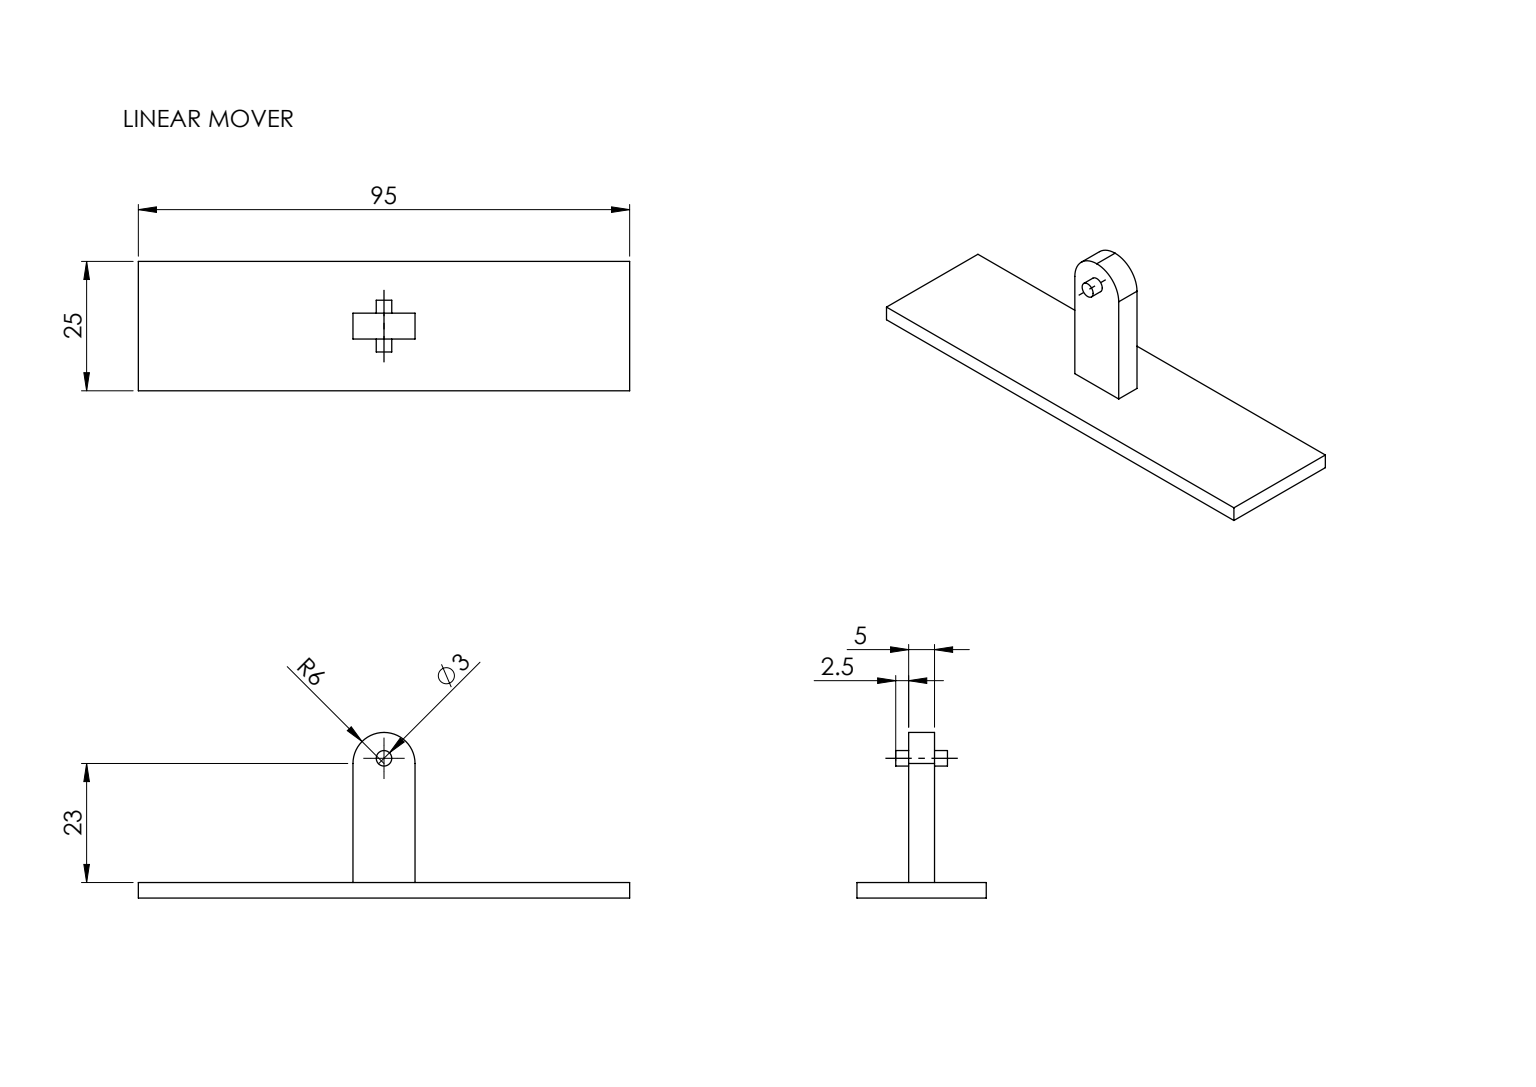
ISO-10303-21;
HEADER;
FILE_DESCRIPTION (('STEP AP214'),
    '1' );
FILE_NAME ('linear mover.step',
    '2026-10-04T07:56:41',
    ( '' ),
    ( '' ),
    'SwSTEP 2.0',
    'SolidWorks 2026',
    '' );
FILE_SCHEMA (( 'AUTOMOTIVE_DESIGN' ));
ENDSEC;

DATA;
#6=DIRECTION ( 'NONE',  ( -1.000000000000000000, 0.000000000000000000, -0.000000000000000000 ) ) ;
#12=EDGE_CURVE ( 'NONE', #8085, #480, #389, .T. ) ;
#26=VERTEX_POINT ( 'NONE', #1027 ) ;
#28=DIRECTION ( 'NONE',  ( 0.000000000000000000, -1.000000000000000000, 0.000000000000000000 ) ) ;
#55=VECTOR ( 'NONE', #6929, 1000.000000000000000 ) ;
#60=CARTESIAN_POINT ( 'NONE',  ( -1.500000000000001110, -27.00000000000000000, 5.000000000000000000 ) ) ;
#65=CARTESIAN_POINT ( 'NONE',  ( -5.999999999999993783, -51.00000000000000711, -2.499999999999999112 ) ) ;
#73=CARTESIAN_POINT ( 'NONE',  ( 3.943604702053941724E-15, -27.99999999999999645, 0.000000000000000000 ) ) ;
#92=CARTESIAN_POINT ( 'NONE',  ( -47.50000000000000711, 47.23441352194253540, 12.50000000000001954 ) ) ;
#102=EDGE_CURVE ( 'NONE', #5844, #6402, #2825, .T. ) ;
#104=DIRECTION ( 'NONE',  ( 0.000000000000000000, -1.000000000000000000, 0.000000000000000000 ) ) ;
#117=CARTESIAN_POINT ( 'NONE',  ( 47.50000000000002132, 47.23441352194253540, 12.50000000000001954 ) ) ;
#151=LINE ( 'NONE', #65, #1132 ) ;
#174=CARTESIAN_POINT ( 'NONE',  ( 1.500000000000002442, -27.00000000000000000, 5.000000000000000000 ) ) ;
#186=EDGE_CURVE ( 'NONE', #2522, #3855, #7004, .T. ) ;
#188=PLANE ( 'NONE',  #457 ) ;
#200=VERTEX_POINT ( 'NONE', #6335 ) ;
#221=ORIENTED_EDGE ( 'NONE', *, *, #2206, .T. ) ;
#222=ADVANCED_FACE ( 'NONE', ( #7515 ), #5686, .T. ) ;
#229=CARTESIAN_POINT ( 'NONE',  ( -5.999999999999993783, -51.00000000000000711, 2.500000000000000888 ) ) ;
#248=ADVANCED_FACE ( 'NONE', ( #3343 ), #5902, .T. ) ;
#294=CARTESIAN_POINT ( 'NONE',  ( 6.123233995736760366E-16, -27.00000000000000000, -5.000000000000000000 ) ) ;
#317=AXIS2_PLACEMENT_3D ( 'NONE', #4788, #4662, #4742 ) ;
#324=ORIENTED_EDGE ( 'NONE', *, *, #6025, .F. ) ;
#334=ORIENTED_EDGE ( 'NONE', *, *, #1098, .F. ) ;
#335=DIRECTION ( 'NONE',  ( 0.000000000000000000, -1.000000000000000000, 0.000000000000000000 ) ) ;
#347=AXIS2_PLACEMENT_3D ( 'NONE', #2756, #5316, #6516 ) ;
#357=LINE ( 'NONE', #7564, #55 ) ;
#376=FACE_OUTER_BOUND ( 'NONE', #2659, .T. ) ;
#389=LINE ( 'NONE', #6796, #1413 ) ;
#404=CARTESIAN_POINT ( 'NONE',  ( 1.500000000000002442, -27.00000000000000000, -5.000000000000000000 ) ) ;
#407=EDGE_CURVE ( 'NONE', #3855, #7622, #7218, .T. ) ;
#457=AXIS2_PLACEMENT_3D ( 'NONE', #229, #7354, #5285 ) ;
#480=VERTEX_POINT ( 'NONE', #1359 ) ;
#494=LINE ( 'NONE', #4888, #7793 ) ;
#505=ORIENTED_EDGE ( 'NONE', *, *, #407, .F. ) ;
#520=EDGE_CURVE ( 'NONE', #5844, #1714, #3390, .T. ) ;
#527=EDGE_CURVE ( 'NONE', #6149, #6264, #3180, .T. ) ;
#560=FILL_AREA_STYLE ('',( #6421 ) ) ;
#583=EDGE_CURVE ( 'NONE', #2431, #1587, #151, .T. ) ;
#601=EDGE_LOOP ( 'NONE', ( #1616, #6343 ) ) ;
#603=CARTESIAN_POINT ( 'NONE',  ( -6.000000000000007994, -51.00000000000000711, -2.499999999999999112 ) ) ;
#631=DIRECTION ( 'NONE',  ( -1.000000000000000000, -9.251858538542971581E-17, 0.000000000000000000 ) ) ;
#634=LINE ( 'NONE', #6416, #4270 ) ;
#643=LINE ( 'NONE', #7606, #1269 ) ;
#644=PLANE ( 'NONE',  #1398 ) ;
#665=CIRCLE ( 'NONE', #6993, 1.500000000000001776 ) ;
#682=CARTESIAN_POINT ( 'NONE',  ( 6.000000000000006217, -51.00000000000000711, -2.499999999999999112 ) ) ;
#718=VECTOR ( 'NONE', #2739, 1000.000000000000000 ) ;
#761=DIRECTION ( 'NONE',  ( -0.000000000000000000, -0.000000000000000000, -1.000000000000000000 ) ) ;
#767=SURFACE_STYLE_USAGE ( .BOTH. , #2128 ) ;
#774=VECTOR ( 'NONE', #3392, 1000.000000000000000 ) ;
#790=AXIS2_PLACEMENT_3D ( 'NONE', #5005, #6189, #6861 ) ;
#798=AXIS2_PLACEMENT_3D ( 'NONE', #4981, #6292, #1833 ) ;
#812=CARTESIAN_POINT ( 'NONE',  ( 47.50000000000002132, -51.00000000000000711, 12.50000000000001954 ) ) ;
#813=DIRECTION ( 'NONE',  ( -0.000000000000000000, 0.000000000000000000, 1.000000000000000000 ) ) ;
#815=( NAMED_UNIT ( * ) PLANE_ANGLE_UNIT ( ) SI_UNIT ( $, .RADIAN. ) );
#819=ORIENTED_EDGE ( 'NONE', *, *, #3574, .T. ) ;
#823=CARTESIAN_POINT ( 'NONE',  ( 6.123233995736760366E-16, -27.00000000000000000, 5.000000000000000000 ) ) ;
#836=EDGE_LOOP ( 'NONE', ( #887, #6399, #4325, #7473 ) ) ;
#853=AXIS2_PLACEMENT_3D ( 'NONE', #1845, #3229, #5871 ) ;
#857=SHAPE_REPRESENTATION_RELATIONSHIP ( 'NONE' , 'NONE' ,  #1989, #7100 ) ;
#860=AXIS2_PLACEMENT_3D ( 'NONE', #117, #1429, #3374 ) ;
#887=ORIENTED_EDGE ( 'NONE', *, *, #186, .T. ) ;
#904=EDGE_LOOP ( 'NONE', ( #7202, #2274, #7512, #7032, #7609 ) ) ;
#928=CARTESIAN_POINT ( 'NONE',  ( 6.000000000000004441, -27.99999999999999645, 2.500000000000000888 ) ) ;
#931=EDGE_CURVE ( 'NONE', #6079, #3352, #634, .T. ) ;
#938=CARTESIAN_POINT ( 'NONE',  ( 6.000000000000006217, -51.00000000000000711, 2.500000000000000888 ) ) ;
#943=VERTEX_POINT ( 'NONE', #2633 ) ;
#979=UNCERTAINTY_MEASURE_WITH_UNIT (LENGTH_MEASURE( 1.000000000000000082E-05 ), #1240, 'distance_accuracy_value', 'NONE');
#996=VERTEX_POINT ( 'NONE', #2046 ) ;
#1027=CARTESIAN_POINT ( 'NONE',  ( -1.500000000000001110, -27.00000000000000000, 2.500000000000000888 ) ) ;
#1073=VECTOR ( 'NONE', #4781, 1000.000000000000000 ) ;
#1079=MECHANICAL_DESIGN_GEOMETRIC_PRESENTATION_REPRESENTATION('',(#5919),#7416);
#1098=EDGE_CURVE ( 'NONE', #2188, #4993, #6582, .T. ) ;
#1111=LINE ( 'NONE', #3683, #4625 ) ;
#1120=LINE ( 'NONE', #1760, #8127 ) ;
#1130=AXIS2_PLACEMENT_3D ( 'NONE', #6423, #2642, #3184 ) ;
#1132=VECTOR ( 'NONE', #7276, 1000.000000000000000 ) ;
#1179=EDGE_LOOP ( 'NONE', ( #5757, #6068, #5152, #5321, #3694 ) ) ;
#1205=PRODUCT_CONTEXT ( 'NONE', #5879, 'mechanical' ) ;
#1219=ORIENTED_EDGE ( 'NONE', *, *, #8239, .T. ) ;
#1222=EDGE_LOOP ( 'NONE', ( #5531, #221 ) ) ;
#1240=( LENGTH_UNIT ( ) NAMED_UNIT ( * ) SI_UNIT ( .MILLI., .METRE. ) );
#1241=VERTEX_POINT ( 'NONE', #8061 ) ;
#1248=FACE_OUTER_BOUND ( 'NONE', #1759, .T. ) ;
#1257=ORIENTED_EDGE ( 'NONE', *, *, #2308, .T. ) ;
#1264=VECTOR ( 'NONE', #28, 1000.000000000000000 ) ;
#1269=VECTOR ( 'NONE', #3226, 1000.000000000000000 ) ;
#1286=DIRECTION ( 'NONE',  ( 1.000000000000000000, 0.000000000000000000, -0.000000000000000000 ) ) ;
#1322=ORIENTED_EDGE ( 'NONE', *, *, #7893, .T. ) ;
#1329=DIRECTION ( 'NONE',  ( 0.000000000000000000, -0.000000000000000000, -1.000000000000000000 ) ) ;
#1338=VECTOR ( 'NONE', #7478, 1000.000000000000000 ) ;
#1359=CARTESIAN_POINT ( 'NONE',  ( 47.50000000000002132, -54.00000000000000711, 12.50000000000001954 ) ) ;
#1366=( LENGTH_UNIT ( ) NAMED_UNIT ( * ) SI_UNIT ( .MILLI., .METRE. ) );
#1372=DIRECTION ( 'NONE',  ( -0.000000000000000000, -0.000000000000000000, 1.000000000000000000 ) ) ;
#1382=FACE_OUTER_BOUND ( 'NONE', #7336, .T. ) ;
#1398=AXIS2_PLACEMENT_3D ( 'NONE', #5158, #2596, #5786 ) ;
#1403=DIRECTION ( 'NONE',  ( -1.000000000000000000, 0.000000000000000000, -0.000000000000000000 ) ) ;
#1413=VECTOR ( 'NONE', #2847, 1000.000000000000000 ) ;
#1429=DIRECTION ( 'NONE',  ( 0.000000000000000000, 0.000000000000000000, 1.000000000000000000 ) ) ;
#1442=DIRECTION ( 'NONE',  ( -0.000000000000000000, -0.000000000000000000, 1.000000000000000000 ) ) ;
#1461=DIRECTION ( 'NONE',  ( 0.000000000000000000, -0.000000000000000000, 1.000000000000000000 ) ) ;
#1469=CARTESIAN_POINT ( 'NONE',  ( -6.000000000000007105, -51.00000000000000711, 2.500000000000000888 ) ) ;
#1518=AXIS2_PLACEMENT_3D ( 'NONE', #682, #3093, #6 ) ;
#1527=DIRECTION ( 'NONE',  ( 1.000000000000000000, -0.000000000000000000, -0.000000000000000000 ) ) ;
#1587=VERTEX_POINT ( 'NONE', #5125 ) ;
#1616=ORIENTED_EDGE ( 'NONE', *, *, #6025, .T. ) ;
#1622=ORIENTED_EDGE ( 'NONE', *, *, #3574, .F. ) ;
#1638=ORIENTED_EDGE ( 'NONE', *, *, #931, .F. ) ;
#1648=PRODUCT_DEFINITION_SHAPE ( 'NONE', 'NONE',  #5608 ) ;
#1714=VERTEX_POINT ( 'NONE', #2229 ) ;
#1754=VECTOR ( 'NONE', #2668, 1000.000000000000000 ) ;
#1756=DIRECTION ( 'NONE',  ( 1.000000000000000000, 0.000000000000000000, 0.000000000000000000 ) ) ;
#1759=EDGE_LOOP ( 'NONE', ( #4728, #819, #2885, #1322 ) ) ;
#1760=CARTESIAN_POINT ( 'NONE',  ( -47.50000000000000711, -54.00000000000000711, 12.50000000000001954 ) ) ;
#1771=CYLINDRICAL_SURFACE ( 'NONE', #790, 1.500000000000001776 ) ;
#1776=EDGE_CURVE ( 'NONE', #7622, #8018, #6521, .T. ) ;
#1788=PRODUCT ( 'linear mover', 'linear mover', '', ( #1205 ) ) ;
#1794=VECTOR ( 'NONE', #1527, 1000.000000000000000 ) ;
#1828=DIRECTION ( 'NONE',  ( 0.000000000000000000, 0.000000000000000000, 1.000000000000000000 ) ) ;
#1833=DIRECTION ( 'NONE',  ( 1.000000000000000000, 0.000000000000000000, 0.000000000000000000 ) ) ;
#1837=ADVANCED_FACE ( 'NONE', ( #7446 ), #2184, .T. ) ;
#1845=CARTESIAN_POINT ( 'NONE',  ( 47.50000000000002132, 47.23441352194253540, 12.50000000000001954 ) ) ;
#1877=FACE_OUTER_BOUND ( 'NONE', #6061, .T. ) ;
#1900=CARTESIAN_POINT ( 'NONE',  ( 3.943604702053941724E-15, -27.99999999999999645, -2.499999999999999112 ) ) ;
#1923=CARTESIAN_POINT ( 'NONE',  ( 4.336808689942017736E-15, -22.00000000000000000, -2.499999999999999112 ) ) ;
#1929=CARTESIAN_POINT ( 'NONE',  ( 4.336808689942017736E-15, -22.00000000000000000, 2.500000000000000888 ) ) ;
#1940=DIRECTION ( 'NONE',  ( 0.000000000000000000, 0.000000000000000000, -1.000000000000000000 ) ) ;
#1981=EDGE_CURVE ( 'NONE', #6079, #943, #357, .T. ) ;
#1984=LINE ( 'NONE', #3707, #5974 ) ;
#1989=SHAPE_REPRESENTATION ( 'linear mover', ( #2840 ), #6190 ) ;
#2012=LINE ( 'NONE', #3190, #2032 ) ;
#2032=VECTOR ( 'NONE', #3902, 1000.000000000000000 ) ;
#2043=CARTESIAN_POINT ( 'NONE',  ( 6.123233995736760366E-16, -27.00000000000000000, 5.000000000000000000 ) ) ;
#2046=CARTESIAN_POINT ( 'NONE',  ( -47.50000000000000711, -51.00000000000000711, 12.50000000000001954 ) ) ;
#2047=LINE ( 'NONE', #2718, #1794 ) ;
#2087=PRESENTATION_STYLE_ASSIGNMENT (( #767 ) ) ;
#2108=LINE ( 'NONE', #5383, #718 ) ;
#2114=VECTOR ( 'NONE', #7899, 1000.000000000000000 ) ;
#2128=SURFACE_SIDE_STYLE ('',( #7818 ) ) ;
#2151=DIRECTION ( 'NONE',  ( -1.000000000000000000, 0.000000000000000000, 0.000000000000000000 ) ) ;
#2184=CYLINDRICAL_SURFACE ( 'NONE', #5842, 6.000000000000000000 ) ;
#2188=VERTEX_POINT ( 'NONE', #6970 ) ;
#2189=CARTESIAN_POINT ( 'NONE',  ( -1.500000000000001110, -27.00000000000000000, 5.000000000000000000 ) ) ;
#2206=EDGE_CURVE ( 'NONE', #4617, #2910, #7590, .T. ) ;
#2229=CARTESIAN_POINT ( 'NONE',  ( 1.500000000000002442, -27.00000000000000000, 2.500000000000000888 ) ) ;
#2235=EDGE_LOOP ( 'NONE', ( #334, #7577, #2698, #5736 ) ) ;
#2254=DIRECTION ( 'NONE',  ( -9.251858538542971581E-17, 1.000000000000000000, 0.000000000000000000 ) ) ;
#2270=ORIENTED_EDGE ( 'NONE', *, *, #7335, .T. ) ;
#2274=ORIENTED_EDGE ( 'NONE', *, *, #6302, .T. ) ;
#2284=DIRECTION ( 'NONE',  ( 1.000000000000000000, 0.000000000000000000, 0.000000000000000000 ) ) ;
#2297=ORIENTED_EDGE ( 'NONE', *, *, #5110, .T. ) ;
#2308=EDGE_CURVE ( 'NONE', #996, #2188, #643, .T. ) ;
#2379=EDGE_CURVE ( 'NONE', #3352, #2522, #2509, .T. ) ;
#2416=AXIS2_PLACEMENT_3D ( 'NONE', #294, #7894, #2911 ) ;
#2431=VERTEX_POINT ( 'NONE', #603 ) ;
#2444=DIRECTION ( 'NONE',  ( -0.000000000000000000, -0.000000000000000000, -1.000000000000000000 ) ) ;
#2454=VERTEX_POINT ( 'NONE', #1923 ) ;
#2472=AXIS2_PLACEMENT_3D ( 'NONE', #938, #5448, #2254 ) ;
#2509=LINE ( 'NONE', #7736, #6911 ) ;
#2522=VERTEX_POINT ( 'NONE', #6550 ) ;
#2544=VECTOR ( 'NONE', #1442, 1000.000000000000000 ) ;
#2554=ADVANCED_FACE ( 'NONE', ( #4064, #3354 ), #188, .T. ) ;
#2555=EDGE_LOOP ( 'NONE', ( #3396, #7430 ) ) ;
#2588=( NAMED_UNIT ( * ) SI_UNIT ( $, .STERADIAN. ) SOLID_ANGLE_UNIT ( ) );
#2592=EDGE_CURVE ( 'NONE', #8018, #943, #7870, .T. ) ;
#2596=DIRECTION ( 'NONE',  ( 0.000000000000000000, 0.000000000000000000, 1.000000000000000000 ) ) ;
#2613=ORIENTED_EDGE ( 'NONE', *, *, #5114, .F. ) ;
#2633=CARTESIAN_POINT ( 'NONE',  ( -5.999999999999995559, -27.99999999999999645, 2.500000000000000888 ) ) ;
#2639=PRESENTATION_STYLE_ASSIGNMENT (( #5821 ) ) ;
#2642=DIRECTION ( 'NONE',  ( -0.000000000000000000, -0.000000000000000000, 1.000000000000000000 ) ) ;
#2659=EDGE_LOOP ( 'NONE', ( #8266, #1257, #5282, #4966 ) ) ;
#2668=DIRECTION ( 'NONE',  ( 0.000000000000000000, 0.000000000000000000, 1.000000000000000000 ) ) ;
#2684=AXIS2_PLACEMENT_3D ( 'NONE', #6539, #631, #3215 ) ;
#2698=ORIENTED_EDGE ( 'NONE', *, *, #12, .F. ) ;
#2718=CARTESIAN_POINT ( 'NONE',  ( 47.50000000000002132, -54.00000000000000711, -12.50000000000001954 ) ) ;
#2738=ORIENTED_EDGE ( 'NONE', *, *, #7893, .F. ) ;
#2739=DIRECTION ( 'NONE',  ( -0.000000000000000000, -0.000000000000000000, -1.000000000000000000 ) ) ;
#2756=CARTESIAN_POINT ( 'NONE',  ( 6.123233995736760366E-16, -27.00000000000000000, -5.000000000000000000 ) ) ;
#2791=DIRECTION ( 'NONE',  ( -0.000000000000000000, 0.000000000000000000, -1.000000000000000000 ) ) ;
#2825=CIRCLE ( 'NONE', #798, 1.500000000000001776 ) ;
#2840=AXIS2_PLACEMENT_3D ( 'NONE', #8120, #5497, #1756 ) ;
#2847=DIRECTION ( 'NONE',  ( -0.000000000000000000, -0.000000000000000000, 1.000000000000000000 ) ) ;
#2880=VECTOR ( 'NONE', #6606, 1000.000000000000000 ) ;
#2885=ORIENTED_EDGE ( 'NONE', *, *, #12, .T. ) ;
#2896=ORIENTED_EDGE ( 'NONE', *, *, #7440, .F. ) ;
#2899=EDGE_LOOP ( 'NONE', ( #7653, #5976, #3115, #7242 ) ) ;
#2903=ORIENTED_EDGE ( 'NONE', *, *, #3156, .T. ) ;
#2910=VERTEX_POINT ( 'NONE', #6168 ) ;
#2911=DIRECTION ( 'NONE',  ( 1.000000000000000000, 0.000000000000000000, 0.000000000000000000 ) ) ;
#2919=EDGE_CURVE ( 'NONE', #4993, #1241, #1111, .T. ) ;
#2920=UNCERTAINTY_MEASURE_WITH_UNIT (LENGTH_MEASURE( 1.000000000000000082E-05 ), #1366, 'distance_accuracy_value', 'NONE');
#2949=ORIENTED_EDGE ( 'NONE', *, *, #102, .F. ) ;
#2950=FACE_OUTER_BOUND ( 'NONE', #7388, .T. ) ;
#2952=DIRECTION ( 'NONE',  ( 0.000000000000000000, -0.000000000000000000, -1.000000000000000000 ) ) ;
#3009=AXIS2_PLACEMENT_3D ( 'NONE', #6469, #7780, #1286 ) ;
#3020=CARTESIAN_POINT ( 'NONE',  ( -1.500000000000001110, -27.00000000000000000, -5.000000000000000000 ) ) ;
#3042=EDGE_LOOP ( 'NONE', ( #6591, #5673, #3523, #2270 ) ) ;
#3093=DIRECTION ( 'NONE',  ( 0.000000000000000000, 0.000000000000000000, -1.000000000000000000 ) ) ;
#3115=ORIENTED_EDGE ( 'NONE', *, *, #6256, .T. ) ;
#3142=ORIENTED_EDGE ( 'NONE', *, *, #7212, .F. ) ;
#3148=ADVANCED_FACE ( 'NONE', ( #5818, #7685 ), #4512, .T. ) ;
#3156=EDGE_CURVE ( 'NONE', #996, #200, #4347, .T. ) ;
#3162=ORIENTED_EDGE ( 'NONE', *, *, #520, .F. ) ;
#3177=DIRECTION ( 'NONE',  ( -0.000000000000000000, 0.000000000000000000, -1.000000000000000000 ) ) ;
#3180=CIRCLE ( 'NONE', #347, 1.500000000000001776 ) ;
#3184=DIRECTION ( 'NONE',  ( -1.000000000000000000, 0.000000000000000000, 0.000000000000000000 ) ) ;
#3190=CARTESIAN_POINT ( 'NONE',  ( 47.50000000000002132, -54.00000000000000711, 12.50000000000001954 ) ) ;
#3215=DIRECTION ( 'NONE',  ( 9.251858538542971581E-17, -1.000000000000000000, 0.000000000000000000 ) ) ;
#3226=DIRECTION ( 'NONE',  ( 1.000000000000000000, 0.000000000000000000, -0.000000000000000000 ) ) ;
#3229=DIRECTION ( 'NONE',  ( 1.000000000000000000, 0.000000000000000000, 0.000000000000000000 ) ) ;
#3262=DIRECTION ( 'NONE',  ( -1.000000000000000000, 0.000000000000000000, 0.000000000000000000 ) ) ;
#3265=SURFACE_SIDE_STYLE ('',( #7648 ) ) ;
#3283=ADVANCED_FACE ( 'NONE', ( #1877 ), #6339, .T. ) ;
#3329=DIRECTION ( 'NONE',  ( -0.000000000000000000, -0.000000000000000000, -1.000000000000000000 ) ) ;
#3343=FACE_OUTER_BOUND ( 'NONE', #2899, .T. ) ;
#3352=VERTEX_POINT ( 'NONE', #8274 ) ;
#3354=FACE_OUTER_BOUND ( 'NONE', #1179, .T. ) ;
#3367=CARTESIAN_POINT ( 'NONE',  ( 3.943604702053941724E-15, -27.99999999999999645, 2.500000000000000888 ) ) ;
#3374=DIRECTION ( 'NONE',  ( 1.000000000000000000, 0.000000000000000000, -0.000000000000000000 ) ) ;
#3390=LINE ( 'NONE', #174, #2114 ) ;
#3392=DIRECTION ( 'NONE',  ( 0.000000000000000000, 0.000000000000000000, -1.000000000000000000 ) ) ;
#3393=FACE_OUTER_BOUND ( 'NONE', #7666, .T. ) ;
#3396=ORIENTED_EDGE ( 'NONE', *, *, #7440, .T. ) ;
#3403=DIRECTION ( 'NONE',  ( -0.000000000000000000, -0.000000000000000000, -1.000000000000000000 ) ) ;
#3414=CYLINDRICAL_SURFACE ( 'NONE', #5691, 1.500000000000001776 ) ;
#3421=VECTOR ( 'NONE', #6765, 1000.000000000000000 ) ;
#3443=LINE ( 'NONE', #7356, #5777 ) ;
#3450=ORIENTED_EDGE ( 'NONE', *, *, #2206, .F. ) ;
#3499=AXIS2_PLACEMENT_3D ( 'NONE', #7376, #335, #2952 ) ;
#3523=ORIENTED_EDGE ( 'NONE', *, *, #583, .F. ) ;
#3574=EDGE_CURVE ( 'NONE', #4272, #8085, #2047, .T. ) ;
#3611=CARTESIAN_POINT ( 'NONE',  ( 3.943604702053941724E-15, -27.99999999999999645, -2.499999999999999112 ) ) ;
#3624=ADVANCED_FACE ( 'NONE', ( #3393 ), #5951, .T. ) ;
#3634=AXIS2_PLACEMENT_3D ( 'NONE', #823, #3403, #7404 ) ;
#3683=CARTESIAN_POINT ( 'NONE',  ( 47.50000000000002132, -51.00000000000000711, -12.50000000000001954 ) ) ;
#3689=COLOUR_RGB ( '', 0.31764706, 0.68627451, 0.89019608) ;
#3694=ORIENTED_EDGE ( 'NONE', *, *, #931, .T. ) ;
#3695=DIRECTION ( 'NONE',  ( -1.000000000000000000, 0.000000000000000000, 0.000000000000000000 ) ) ;
#3707=CARTESIAN_POINT ( 'NONE',  ( -5.999999999999995559, -27.99999999999999645, -2.499999999999999112 ) ) ;
#3747=EDGE_LOOP ( 'NONE', ( #2949, #8139, #324, #5581 ) ) ;
#3768=EDGE_CURVE ( 'NONE', #2188, #480, #7428, .T. ) ;
#3813=SHAPE_DEFINITION_REPRESENTATION ( #1648, #1989 ) ;
#3816=PLANE ( 'NONE',  #853 ) ;
#3855=VERTEX_POINT ( 'NONE', #7344 ) ;
#3868=ORIENTED_EDGE ( 'NONE', *, *, #5110, .F. ) ;
#3870=LINE ( 'NONE', #5799, #1264 ) ;
#3902=DIRECTION ( 'NONE',  ( -1.000000000000000000, 0.000000000000000000, 0.000000000000000000 ) ) ;
#3925=CARTESIAN_POINT ( 'NONE',  ( 6.123233995736760366E-16, -27.00000000000000000, 5.000000000000000000 ) ) ;
#3990=DIRECTION ( 'NONE',  ( 1.000000000000000000, 0.000000000000000000, 0.000000000000000000 ) ) ;
#4015=( LENGTH_UNIT ( ) NAMED_UNIT ( * ) SI_UNIT ( .MILLI., .METRE. ) );
#4061=( NAMED_UNIT ( * ) SI_UNIT ( $, .STERADIAN. ) SOLID_ANGLE_UNIT ( ) );
#4064=FACE_BOUND ( 'NONE', #601, .T. ) ;
#4086=EDGE_CURVE ( 'NONE', #1241, #4272, #3870, .T. ) ;
#4088=EDGE_CURVE ( 'NONE', #943, #1587, #1984, .T. ) ;
#4094=VECTOR ( 'NONE', #1828, 1000.000000000000000 ) ;
#4127=CARTESIAN_POINT ( 'NONE',  ( 6.123233995736760366E-16, -27.00000000000000000, 2.500000000000000888 ) ) ;
#4138=ADVANCED_FACE ( 'NONE', ( #5716 ), #8295, .T. ) ;
#4152=ORIENTED_EDGE ( 'NONE', *, *, #2379, .F. ) ;
#4153=CIRCLE ( 'NONE', #2416, 1.500000000000001776 ) ;
#4209=PLANE ( 'NONE',  #3499 ) ;
#4225=ORIENTED_EDGE ( 'NONE', *, *, #4086, .F. ) ;
#4266=DIRECTION ( 'NONE',  ( -1.000000000000000000, 0.000000000000000000, 0.000000000000000000 ) ) ;
#4267=ADVANCED_FACE ( 'NONE', ( #5259 ), #3414, .T. ) ;
#4270=VECTOR ( 'NONE', #5817, 1000.000000000000000 ) ;
#4272=VERTEX_POINT ( 'NONE', #5887 ) ;
#4325=ORIENTED_EDGE ( 'NONE', *, *, #6898, .F. ) ;
#4338=ORIENTED_EDGE ( 'NONE', *, *, #2919, .F. ) ;
#4347=LINE ( 'NONE', #7727, #4737 ) ;
#4378=MANIFOLD_SOLID_BREP ( 'Boss-Extrude4', #5181 ) ;
#4391=ORIENTED_EDGE ( 'NONE', *, *, #1776, .F. ) ;
#4426=CIRCLE ( 'NONE', #4840, 1.500000000000001776 ) ;
#4460=ADVANCED_FACE ( 'NONE', ( #7303 ), #6705, .T. ) ;
#4482=PLANE ( 'NONE',  #6462 ) ;
#4512=PLANE ( 'NONE',  #1518 ) ;
#4578=ORIENTED_EDGE ( 'NONE', *, *, #7335, .F. ) ;
#4599=( NAMED_UNIT ( * ) PLANE_ANGLE_UNIT ( ) SI_UNIT ( $, .RADIAN. ) );
#4602=DIRECTION ( 'NONE',  ( 1.000000000000000000, 0.000000000000000000, 0.000000000000000000 ) ) ;
#4617=VERTEX_POINT ( 'NONE', #8147 ) ;
#4625=VECTOR ( 'NONE', #4266, 1000.000000000000000 ) ;
#4652=CARTESIAN_POINT ( 'NONE',  ( 47.50000000000002132, -54.00000000000000711, -12.50000000000001954 ) ) ;
#4662=DIRECTION ( 'NONE',  ( -0.000000000000000000, 0.000000000000000000, -1.000000000000000000 ) ) ;
#4680=( NAMED_UNIT ( * ) SI_UNIT ( $, .STERADIAN. ) SOLID_ANGLE_UNIT ( ) );
#4724=ORIENTED_EDGE ( 'NONE', *, *, #6060, .T. ) ;
#4728=ORIENTED_EDGE ( 'NONE', *, *, #6341, .T. ) ;
#4737=VECTOR ( 'NONE', #7644, 1000.000000000000000 ) ;
#4742=DIRECTION ( 'NONE',  ( 1.000000000000000000, 0.000000000000000000, 0.000000000000000000 ) ) ;
#4781=DIRECTION ( 'NONE',  ( 0.000000000000000000, -0.000000000000000000, 1.000000000000000000 ) ) ;
#4788=CARTESIAN_POINT ( 'NONE',  ( 6.123233995736760366E-16, -27.00000000000000000, 2.500000000000000888 ) ) ;
#4822=FACE_OUTER_BOUND ( 'NONE', #7542, .T. ) ;
#4826=CARTESIAN_POINT ( 'NONE',  ( 3.943604702053941724E-15, -27.99999999999999645, 0.000000000000000000 ) ) ;
#4840=AXIS2_PLACEMENT_3D ( 'NONE', #3925, #5225, #5945 ) ;
#4888=CARTESIAN_POINT ( 'NONE',  ( 6.000000000000006217, -51.00000000000000711, -2.499999999999999112 ) ) ;
#4963=CIRCLE ( 'NONE', #5632, 6.000000000000000000 ) ;
#4966=ORIENTED_EDGE ( 'NONE', *, *, #2919, .T. ) ;
#4981=CARTESIAN_POINT ( 'NONE',  ( 6.123233995736760366E-16, -27.00000000000000000, 5.000000000000000000 ) ) ;
#4993=VERTEX_POINT ( 'NONE', #6027 ) ;
#5005=CARTESIAN_POINT ( 'NONE',  ( 6.123233995736760366E-16, -27.00000000000000000, 5.000000000000000000 ) ) ;
#5036=PLANE ( 'NONE',  #3009 ) ;
#5050=ORIENTED_EDGE ( 'NONE', *, *, #5995, .T. ) ;
#5110=EDGE_CURVE ( 'NONE', #6264, #6149, #4153, .T. ) ;
#5114=EDGE_CURVE ( 'NONE', #1714, #26, #8197, .T. ) ;
#5125=CARTESIAN_POINT ( 'NONE',  ( -5.999999999999995559, -27.99999999999999645, -2.499999999999999112 ) ) ;
#5129=DIRECTION ( 'NONE',  ( 0.000000000000000000, 0.000000000000000000, -1.000000000000000000 ) ) ;
#5139=CARTESIAN_POINT ( 'NONE',  ( -5.999999999999993783, -51.00000000000000711, -2.499999999999999112 ) ) ;
#5150=FILL_AREA_STYLE_COLOUR ( '', #3689 ) ;
#5152=ORIENTED_EDGE ( 'NONE', *, *, #2592, .T. ) ;
#5158=CARTESIAN_POINT ( 'NONE',  ( 6.123233995736760366E-16, -27.00000000000000000, 5.000000000000000000 ) ) ;
#5161=CARTESIAN_POINT ( 'NONE',  ( 0.000000000000000000, -54.00000000000000711, 0.000000000000000000 ) ) ;
#5172=DIRECTION ( 'NONE',  ( -1.000000000000000000, 0.000000000000000000, 0.000000000000000000 ) ) ;
#5181=CLOSED_SHELL ( 'NONE', ( #8149, #4267, #222, #3148, #4460, #2554, #1837, #5537, #6675, #5403, #248, #6391, #7690, #3624, #4138, #6586, #3283, #7847 ) ) ;
#5186=LINE ( 'NONE', #5139, #1754 ) ;
#5200=FACE_OUTER_BOUND ( 'NONE', #2235, .T. ) ;
#5214=DIRECTION ( 'NONE',  ( -1.000000000000000000, 0.000000000000000000, 0.000000000000000000 ) ) ;
#5225=DIRECTION ( 'NONE',  ( 0.000000000000000000, 0.000000000000000000, 1.000000000000000000 ) ) ;
#5229=DIRECTION ( 'NONE',  ( -1.000000000000000000, 0.000000000000000000, 0.000000000000000000 ) ) ;
#5240=CARTESIAN_POINT ( 'NONE',  ( 3.943604702053941724E-15, -27.99999999999999645, 2.500000000000000888 ) ) ;
#5253=COLOUR_RGB ( '', 0.31764706, 0.68627451, 0.89019608) ;
#5259=FACE_OUTER_BOUND ( 'NONE', #3747, .T. ) ;
#5282=ORIENTED_EDGE ( 'NONE', *, *, #1098, .T. ) ;
#5285=DIRECTION ( 'NONE',  ( 1.000000000000000000, 0.000000000000000000, -0.000000000000000000 ) ) ;
#5307=AXIS2_PLACEMENT_3D ( 'NONE', #5240, #7952, #4602 ) ;
#5316=DIRECTION ( 'NONE',  ( 0.000000000000000000, 0.000000000000000000, 1.000000000000000000 ) ) ;
#5321=ORIENTED_EDGE ( 'NONE', *, *, #1981, .F. ) ;
#5326=EDGE_CURVE ( 'NONE', #2522, #2431, #494, .T. ) ;
#5331=DIRECTION ( 'NONE',  ( 0.000000000000000000, -1.000000000000000000, 0.000000000000000000 ) ) ;
#5383=CARTESIAN_POINT ( 'NONE',  ( 1.500000000000002442, -27.00000000000000000, 5.000000000000000000 ) ) ;
#5403=ADVANCED_FACE ( 'NONE', ( #2950 ), #1771, .T. ) ;
#5421=ORIENTED_EDGE ( 'NONE', *, *, #6256, .F. ) ;
#5448=DIRECTION ( 'NONE',  ( 1.000000000000000000, 9.251858538542971581E-17, 0.000000000000000000 ) ) ;
#5464=ORIENTED_EDGE ( 'NONE', *, *, #527, .F. ) ;
#5497=DIRECTION ( 'NONE',  ( 0.000000000000000000, 0.000000000000000000, 1.000000000000000000 ) ) ;
#5531=ORIENTED_EDGE ( 'NONE', *, *, #7898, .T. ) ;
#5537=ADVANCED_FACE ( 'NONE', ( #1382 ), #5886, .T. ) ;
#5544=LINE ( 'NONE', #6136, #3421 ) ;
#5579=ORIENTED_EDGE ( 'NONE', *, *, #3156, .F. ) ;
#5581=ORIENTED_EDGE ( 'NONE', *, *, #6060, .F. ) ;
#5582=DIRECTION ( 'NONE',  ( 0.000000000000000000, 0.000000000000000000, -1.000000000000000000 ) ) ;
#5597=EDGE_CURVE ( 'NONE', #1587, #2454, #4963, .T. ) ;
#5604=EDGE_LOOP ( 'NONE', ( #6321, #2903, #2738, #6792 ) ) ;
#5608=PRODUCT_DEFINITION ( 'UNKNOWN', '', #6848, #6704 ) ;
#5618=DIRECTION ( 'NONE',  ( 0.000000000000000000, 0.000000000000000000, 1.000000000000000000 ) ) ;
#5632=AXIS2_PLACEMENT_3D ( 'NONE', #1900, #1940, #5172 ) ;
#5673=ORIENTED_EDGE ( 'NONE', *, *, #4088, .T. ) ;
#5683=CARTESIAN_POINT ( 'NONE',  ( -47.50000000000000711, -51.00000000000000711, 12.50000000000001954 ) ) ;
#5686=PLANE ( 'NONE',  #2684 ) ;
#5691=AXIS2_PLACEMENT_3D ( 'NONE', #7204, #3329, #2151 ) ;
#5696=EDGE_LOOP ( 'NONE', ( #5464, #3868 ) ) ;
#5716=FACE_OUTER_BOUND ( 'NONE', #5604, .T. ) ;
#5736=ORIENTED_EDGE ( 'NONE', *, *, #8239, .F. ) ;
#5757=ORIENTED_EDGE ( 'NONE', *, *, #6898, .T. ) ;
#5777=VECTOR ( 'NONE', #5331, 1000.000000000000000 ) ;
#5786=DIRECTION ( 'NONE',  ( 1.000000000000000000, 0.000000000000000000, -0.000000000000000000 ) ) ;
#5799=CARTESIAN_POINT ( 'NONE',  ( -47.50000000000000711, 47.23441352194253540, -12.50000000000001954 ) ) ;
#5817=DIRECTION ( 'NONE',  ( 1.000000000000000000, 0.000000000000000000, 0.000000000000000000 ) ) ;
#5818=FACE_BOUND ( 'NONE', #1222, .T. ) ;
#5821=SURFACE_STYLE_USAGE ( .BOTH. , #3265 ) ;
#5842=AXIS2_PLACEMENT_3D ( 'NONE', #4826, #5618, #8082 ) ;
#5844=VERTEX_POINT ( 'NONE', #6360 ) ;
#5859=CARTESIAN_POINT ( 'NONE',  ( 6.000000000000004441, -27.99999999999999645, 2.500000000000000888 ) ) ;
#5871=DIRECTION ( 'NONE',  ( 0.000000000000000000, 0.000000000000000000, -1.000000000000000000 ) ) ;
#5879=APPLICATION_CONTEXT ( 'automotive_design' ) ;
#5886=CYLINDRICAL_SURFACE ( 'NONE', #7525, 6.000000000000000000 ) ;
#5887=CARTESIAN_POINT ( 'NONE',  ( -47.50000000000000711, -54.00000000000000711, -12.50000000000001954 ) ) ;
#5902=CYLINDRICAL_SURFACE ( 'NONE', #6983, 1.500000000000001776 ) ;
#5919=STYLED_ITEM ( 'NONE', ( #2639 ), #7100 ) ;
#5945=DIRECTION ( 'NONE',  ( 1.000000000000000000, 0.000000000000000000, 0.000000000000000000 ) ) ;
#5951=PLANE ( 'NONE',  #6495 ) ;
#5964=LINE ( 'NONE', #6635, #1073 ) ;
#5974=VECTOR ( 'NONE', #2444, 1000.000000000000000 ) ;
#5976=ORIENTED_EDGE ( 'NONE', *, *, #7898, .F. ) ;
#5977=LINE ( 'NONE', #2189, #2880 ) ;
#5995=EDGE_CURVE ( 'NONE', #4617, #6264, #2108, .T. ) ;
#6025=EDGE_CURVE ( 'NONE', #26, #1714, #7044, .T. ) ;
#6026=EDGE_LOOP ( 'NONE', ( #4578, #6504, #4152, #1638 ) ) ;
#6027=CARTESIAN_POINT ( 'NONE',  ( 47.50000000000002132, -51.00000000000000711, -12.50000000000001954 ) ) ;
#6060=EDGE_CURVE ( 'NONE', #6402, #26, #5977, .T. ) ;
#6061=EDGE_LOOP ( 'NONE', ( #4338, #1219, #1622, #4225 ) ) ;
#6068=ORIENTED_EDGE ( 'NONE', *, *, #1776, .T. ) ;
#6079=VERTEX_POINT ( 'NONE', #1469 ) ;
#6136=CARTESIAN_POINT ( 'NONE',  ( -1.500000000000001110, -27.00000000000000000, 5.000000000000000000 ) ) ;
#6149=VERTEX_POINT ( 'NONE', #3020 ) ;
#6161=DIRECTION ( 'NONE',  ( -9.251858538542971581E-17, 1.000000000000000000, 0.000000000000000000 ) ) ;
#6168=CARTESIAN_POINT ( 'NONE',  ( -1.500000000000001110, -27.00000000000000000, -2.499999999999999556 ) ) ;
#6189=DIRECTION ( 'NONE',  ( -0.000000000000000000, -0.000000000000000000, -1.000000000000000000 ) ) ;
#6190=( GEOMETRIC_REPRESENTATION_CONTEXT ( 3 ) GLOBAL_UNCERTAINTY_ASSIGNED_CONTEXT ( ( #979 ) ) GLOBAL_UNIT_ASSIGNED_CONTEXT ( ( #1240, #8318, #2588 ) ) REPRESENTATION_CONTEXT ( 'NONE', 'WORKASPACE' ) );
#6215=UNCERTAINTY_MEASURE_WITH_UNIT (LENGTH_MEASURE( 1.000000000000000082E-05 ), #4015, 'distance_accuracy_value', 'NONE');
#6245=ORIENTED_EDGE ( 'NONE', *, *, #6341, .F. ) ;
#6246=LINE ( 'NONE', #5683, #4094 ) ;
#6256=EDGE_CURVE ( 'NONE', #2910, #6149, #5544, .T. ) ;
#6264=VERTEX_POINT ( 'NONE', #404 ) ;
#6292=DIRECTION ( 'NONE',  ( 0.000000000000000000, 0.000000000000000000, 1.000000000000000000 ) ) ;
#6302=EDGE_CURVE ( 'NONE', #2454, #3855, #7999, .T. ) ;
#6309=AXIS2_PLACEMENT_3D ( 'NONE', #4127, #2791, #2284 ) ;
#6321=ORIENTED_EDGE ( 'NONE', *, *, #2308, .F. ) ;
#6335=CARTESIAN_POINT ( 'NONE',  ( -47.50000000000000711, -54.00000000000000711, 12.50000000000001954 ) ) ;
#6339=PLANE ( 'NONE',  #6912 ) ;
#6341=EDGE_CURVE ( 'NONE', #200, #4272, #1120, .T. ) ;
#6343=ORIENTED_EDGE ( 'NONE', *, *, #5114, .T. ) ;
#6360=CARTESIAN_POINT ( 'NONE',  ( 1.500000000000002442, -27.00000000000000000, 5.000000000000000000 ) ) ;
#6379=VECTOR ( 'NONE', #6161, 1000.000000000000000 ) ;
#6391=ADVANCED_FACE ( 'NONE', ( #8163 ), #5036, .F. ) ;
#6399=ORIENTED_EDGE ( 'NONE', *, *, #407, .T. ) ;
#6402=VERTEX_POINT ( 'NONE', #60 ) ;
#6416=CARTESIAN_POINT ( 'NONE',  ( -5.999999999999993783, -51.00000000000000711, 2.500000000000000888 ) ) ;
#6421=FILL_AREA_STYLE_COLOUR ( '', #5253 ) ;
#6423=CARTESIAN_POINT ( 'NONE',  ( 6.123233995736760366E-16, -27.00000000000000000, -2.499999999999999556 ) ) ;
#6462=AXIS2_PLACEMENT_3D ( 'NONE', #5161, #104, #1329 ) ;
#6469=CARTESIAN_POINT ( 'NONE',  ( 6.123233995736760366E-16, -27.00000000000000000, -5.000000000000000000 ) ) ;
#6484=EDGE_LOOP ( 'NONE', ( #6647, #6726, #6899, #8100 ) ) ;
#6495=AXIS2_PLACEMENT_3D ( 'NONE', #92, #1403, #813 ) ;
#6504=ORIENTED_EDGE ( 'NONE', *, *, #5326, .F. ) ;
#6513=CARTESIAN_POINT ( 'NONE',  ( 6.123233995736760366E-16, -27.00000000000000000, -2.499999999999999556 ) ) ;
#6516=DIRECTION ( 'NONE',  ( 1.000000000000000000, 0.000000000000000000, 0.000000000000000000 ) ) ;
#6521=CIRCLE ( 'NONE', #7600, 6.000000000000000000 ) ;
#6539=CARTESIAN_POINT ( 'NONE',  ( -5.999999999999993783, -51.00000000000000711, -2.499999999999999112 ) ) ;
#6550=CARTESIAN_POINT ( 'NONE',  ( 6.000000000000006217, -51.00000000000000711, -2.500000000000001776 ) ) ;
#6582=LINE ( 'NONE', #812, #774 ) ;
#6586=ADVANCED_FACE ( 'NONE', ( #5200 ), #3816, .T. ) ;
#6591=ORIENTED_EDGE ( 'NONE', *, *, #1981, .T. ) ;
#6597=CYLINDRICAL_SURFACE ( 'NONE', #3634, 1.500000000000001776 ) ;
#6606=DIRECTION ( 'NONE',  ( -0.000000000000000000, -0.000000000000000000, -1.000000000000000000 ) ) ;
#6635=CARTESIAN_POINT ( 'NONE',  ( 3.943604702053941724E-15, -22.00000000000000000, 0.000000000000000000 ) ) ;
#6647=ORIENTED_EDGE ( 'NONE', *, *, #4088, .F. ) ;
#6660=FACE_BOUND ( 'NONE', #6026, .T. ) ;
#6675=ADVANCED_FACE ( 'NONE', ( #7059 ), #644, .T. ) ;
#6704=PRODUCT_DEFINITION_CONTEXT ( 'detailed design', #7181, 'design' ) ;
#6705=PLANE ( 'NONE',  #2472 ) ;
#6726=ORIENTED_EDGE ( 'NONE', *, *, #2592, .F. ) ;
#6747=DIRECTION ( 'NONE',  ( 0.000000000000000000, -1.000000000000000000, 0.000000000000000000 ) ) ;
#6750=LINE ( 'NONE', #7190, #6379 ) ;
#6765=DIRECTION ( 'NONE',  ( -0.000000000000000000, -0.000000000000000000, -1.000000000000000000 ) ) ;
#6792=ORIENTED_EDGE ( 'NONE', *, *, #3768, .F. ) ;
#6796=CARTESIAN_POINT ( 'NONE',  ( 47.50000000000002132, -54.00000000000000711, 12.50000000000001954 ) ) ;
#6848=PRODUCT_DEFINITION_FORMATION_WITH_SPECIFIED_SOURCE ( 'ANY', '', #1788, .NOT_KNOWN. ) ;
#6861=DIRECTION ( 'NONE',  ( -1.000000000000000000, 0.000000000000000000, 0.000000000000000000 ) ) ;
#6898=EDGE_CURVE ( 'NONE', #3352, #7622, #6750, .T. ) ;
#6899=ORIENTED_EDGE ( 'NONE', *, *, #8173, .F. ) ;
#6911=VECTOR ( 'NONE', #8238, 1000.000000000000000 ) ;
#6912=AXIS2_PLACEMENT_3D ( 'NONE', #7560, #3177, #3262 ) ;
#6929=DIRECTION ( 'NONE',  ( -9.251858538542971581E-17, 1.000000000000000000, 0.000000000000000000 ) ) ;
#6970=CARTESIAN_POINT ( 'NONE',  ( 47.50000000000002132, -51.00000000000000711, 12.50000000000001954 ) ) ;
#6983=AXIS2_PLACEMENT_3D ( 'NONE', #2043, #761, #5229 ) ;
#6988=DIRECTION ( 'NONE',  ( -1.000000000000000000, 0.000000000000000000, 0.000000000000000000 ) ) ;
#6993=AXIS2_PLACEMENT_3D ( 'NONE', #6513, #1372, #7062 ) ;
#7004=LINE ( 'NONE', #7556, #1338 ) ;
#7032=ORIENTED_EDGE ( 'NONE', *, *, #5326, .T. ) ;
#7044=CIRCLE ( 'NONE', #317, 1.500000000000001776 ) ;
#7050=STYLED_ITEM ( 'NONE', ( #2087 ), #4378 ) ;
#7059=FACE_OUTER_BOUND ( 'NONE', #2555, .T. ) ;
#7062=DIRECTION ( 'NONE',  ( -1.000000000000000000, 0.000000000000000000, 0.000000000000000000 ) ) ;
#7100=ADVANCED_BREP_SHAPE_REPRESENTATION ( '', ( #4378, #2840 ), #6190 ) ;
#7180=FILL_AREA_STYLE ('',( #5150 ) ) ;
#7181=APPLICATION_CONTEXT ( 'automotive_design' ) ;
#7190=CARTESIAN_POINT ( 'NONE',  ( 6.000000000000006217, -51.00000000000000711, 2.500000000000000888 ) ) ;
#7202=ORIENTED_EDGE ( 'NONE', *, *, #5597, .T. ) ;
#7204=CARTESIAN_POINT ( 'NONE',  ( 6.123233995736760366E-16, -27.00000000000000000, 5.000000000000000000 ) ) ;
#7212=EDGE_CURVE ( 'NONE', #1241, #996, #6246, .T. ) ;
#7218=LINE ( 'NONE', #5859, #2544 ) ;
#7242=ORIENTED_EDGE ( 'NONE', *, *, #527, .T. ) ;
#7276=DIRECTION ( 'NONE',  ( -9.251858538542971581E-17, 1.000000000000000000, 0.000000000000000000 ) ) ;
#7303=FACE_OUTER_BOUND ( 'NONE', #836, .T. ) ;
#7314=MECHANICAL_DESIGN_GEOMETRIC_PRESENTATION_REPRESENTATION('',(#7050),#7867);
#7335=EDGE_CURVE ( 'NONE', #2431, #6079, #5186, .T. ) ;
#7336=EDGE_LOOP ( 'NONE', ( #4391, #505, #7461, #8278 ) ) ;
#7344=CARTESIAN_POINT ( 'NONE',  ( 6.000000000000004441, -27.99999999999999645, -2.499999999999999112 ) ) ;
#7354=DIRECTION ( 'NONE',  ( 0.000000000000000000, -0.000000000000000000, 1.000000000000000000 ) ) ;
#7356=CARTESIAN_POINT ( 'NONE',  ( 47.50000000000002132, 47.23441352194253540, -12.50000000000001954 ) ) ;
#7376=CARTESIAN_POINT ( 'NONE',  ( 0.000000000000000000, -51.00000000000000711, 0.000000000000000000 ) ) ;
#7388=EDGE_LOOP ( 'NONE', ( #3162, #2896, #4724, #2613 ) ) ;
#7404=DIRECTION ( 'NONE',  ( -1.000000000000000000, 0.000000000000000000, 0.000000000000000000 ) ) ;
#7416=( GEOMETRIC_REPRESENTATION_CONTEXT ( 3 ) GLOBAL_UNCERTAINTY_ASSIGNED_CONTEXT ( ( #2920 ) ) GLOBAL_UNIT_ASSIGNED_CONTEXT ( ( #1366, #4599, #4061 ) ) REPRESENTATION_CONTEXT ( 'NONE', 'WORKASPACE' ) );
#7428=LINE ( 'NONE', #7470, #7457 ) ;
#7430=ORIENTED_EDGE ( 'NONE', *, *, #102, .T. ) ;
#7440=EDGE_CURVE ( 'NONE', #6402, #5844, #4426, .T. ) ;
#7446=FACE_OUTER_BOUND ( 'NONE', #6484, .T. ) ;
#7457=VECTOR ( 'NONE', #6747, 1000.000000000000000 ) ;
#7461=ORIENTED_EDGE ( 'NONE', *, *, #6302, .F. ) ;
#7470=CARTESIAN_POINT ( 'NONE',  ( 47.50000000000002132, 47.23441352194253540, 12.50000000000001954 ) ) ;
#7473=ORIENTED_EDGE ( 'NONE', *, *, #2379, .T. ) ;
#7478=DIRECTION ( 'NONE',  ( -9.251858538542971581E-17, 1.000000000000000000, 0.000000000000000000 ) ) ;
#7512=ORIENTED_EDGE ( 'NONE', *, *, #186, .F. ) ;
#7515=FACE_OUTER_BOUND ( 'NONE', #3042, .T. ) ;
#7525=AXIS2_PLACEMENT_3D ( 'NONE', #73, #5129, #5214 ) ;
#7542=EDGE_LOOP ( 'NONE', ( #3450, #5050, #2297, #5421 ) ) ;
#7556=CARTESIAN_POINT ( 'NONE',  ( 6.000000000000006217, -51.00000000000000711, -2.499999999999999112 ) ) ;
#7560=CARTESIAN_POINT ( 'NONE',  ( 47.50000000000002132, 47.23441352194253540, -12.50000000000001954 ) ) ;
#7564=CARTESIAN_POINT ( 'NONE',  ( -5.999999999999993783, -51.00000000000000711, 2.500000000000000888 ) ) ;
#7566=DIRECTION ( 'NONE',  ( 0.000000000000000000, 0.000000000000000000, -1.000000000000000000 ) ) ;
#7577=ORIENTED_EDGE ( 'NONE', *, *, #3768, .T. ) ;
#7585=AXIS2_PLACEMENT_3D ( 'NONE', #3611, #7566, #3695 ) ;
#7590=CIRCLE ( 'NONE', #1130, 1.500000000000001776 ) ;
#7600=AXIS2_PLACEMENT_3D ( 'NONE', #3367, #1461, #3990 ) ;
#7606=CARTESIAN_POINT ( 'NONE',  ( 47.50000000000002132, -51.00000000000000711, 12.50000000000001954 ) ) ;
#7609=ORIENTED_EDGE ( 'NONE', *, *, #583, .T. ) ;
#7622=VERTEX_POINT ( 'NONE', #928 ) ;
#7644=DIRECTION ( 'NONE',  ( 0.000000000000000000, -1.000000000000000000, 0.000000000000000000 ) ) ;
#7648=SURFACE_STYLE_FILL_AREA ( #560 ) ;
#7653=ORIENTED_EDGE ( 'NONE', *, *, #5995, .F. ) ;
#7666=EDGE_LOOP ( 'NONE', ( #3142, #7974, #6245, #5579 ) ) ;
#7685=FACE_OUTER_BOUND ( 'NONE', #904, .T. ) ;
#7690=ADVANCED_FACE ( 'NONE', ( #6660, #376 ), #4209, .F. ) ;
#7727=CARTESIAN_POINT ( 'NONE',  ( -47.50000000000000711, 47.23441352194253540, 12.50000000000001954 ) ) ;
#7736=CARTESIAN_POINT ( 'NONE',  ( 6.000000000000006217, -51.00000000000000711, 2.500000000000000888 ) ) ;
#7780=DIRECTION ( 'NONE',  ( 0.000000000000000000, 0.000000000000000000, 1.000000000000000000 ) ) ;
#7793=VECTOR ( 'NONE', #6988, 1000.000000000000000 ) ;
#7818=SURFACE_STYLE_FILL_AREA ( #7180 ) ;
#7847=ADVANCED_FACE ( 'NONE', ( #1248 ), #4482, .T. ) ;
#7867=( GEOMETRIC_REPRESENTATION_CONTEXT ( 3 ) GLOBAL_UNCERTAINTY_ASSIGNED_CONTEXT ( ( #6215 ) ) GLOBAL_UNIT_ASSIGNED_CONTEXT ( ( #4015, #815, #4680 ) ) REPRESENTATION_CONTEXT ( 'NONE', 'WORKASPACE' ) );
#7870=CIRCLE ( 'NONE', #5307, 6.000000000000000000 ) ;
#7893=EDGE_CURVE ( 'NONE', #480, #200, #2012, .T. ) ;
#7894=DIRECTION ( 'NONE',  ( 0.000000000000000000, 0.000000000000000000, 1.000000000000000000 ) ) ;
#7898=EDGE_CURVE ( 'NONE', #2910, #4617, #665, .T. ) ;
#7899=DIRECTION ( 'NONE',  ( -0.000000000000000000, -0.000000000000000000, -1.000000000000000000 ) ) ;
#7952=DIRECTION ( 'NONE',  ( 0.000000000000000000, -0.000000000000000000, 1.000000000000000000 ) ) ;
#7974=ORIENTED_EDGE ( 'NONE', *, *, #4086, .T. ) ;
#7999=CIRCLE ( 'NONE', #7585, 6.000000000000000000 ) ;
#8018=VERTEX_POINT ( 'NONE', #1929 ) ;
#8061=CARTESIAN_POINT ( 'NONE',  ( -47.50000000000000711, -51.00000000000000711, -12.50000000000001954 ) ) ;
#8082=DIRECTION ( 'NONE',  ( 1.000000000000000000, 0.000000000000000000, 0.000000000000000000 ) ) ;
#8085=VERTEX_POINT ( 'NONE', #4652 ) ;
#8100=ORIENTED_EDGE ( 'NONE', *, *, #5597, .F. ) ;
#8120=CARTESIAN_POINT ( 'NONE',  ( 0.000000000000000000, 0.000000000000000000, 0.000000000000000000 ) ) ;
#8127=VECTOR ( 'NONE', #5582, 1000.000000000000000 ) ;
#8139=ORIENTED_EDGE ( 'NONE', *, *, #520, .T. ) ;
#8147=CARTESIAN_POINT ( 'NONE',  ( 1.500000000000002442, -27.00000000000000000, -2.499999999999999556 ) ) ;
#8149=ADVANCED_FACE ( 'NONE', ( #4822 ), #6597, .T. ) ;
#8163=FACE_OUTER_BOUND ( 'NONE', #5696, .T. ) ;
#8173=EDGE_CURVE ( 'NONE', #2454, #8018, #5964, .T. ) ;
#8197=CIRCLE ( 'NONE', #6309, 1.500000000000001776 ) ;
#8238=DIRECTION ( 'NONE',  ( 0.000000000000000000, 0.000000000000000000, -1.000000000000000000 ) ) ;
#8239=EDGE_CURVE ( 'NONE', #4993, #8085, #3443, .T. ) ;
#8266=ORIENTED_EDGE ( 'NONE', *, *, #7212, .T. ) ;
#8274=CARTESIAN_POINT ( 'NONE',  ( 6.000000000000006217, -51.00000000000000711, 2.500000000000000888 ) ) ;
#8278=ORIENTED_EDGE ( 'NONE', *, *, #8173, .T. ) ;
#8295=PLANE ( 'NONE',  #860 ) ;
#8318=( NAMED_UNIT ( * ) PLANE_ANGLE_UNIT ( ) SI_UNIT ( $, .RADIAN. ) );
ENDSEC;
END-ISO-10303-21;
